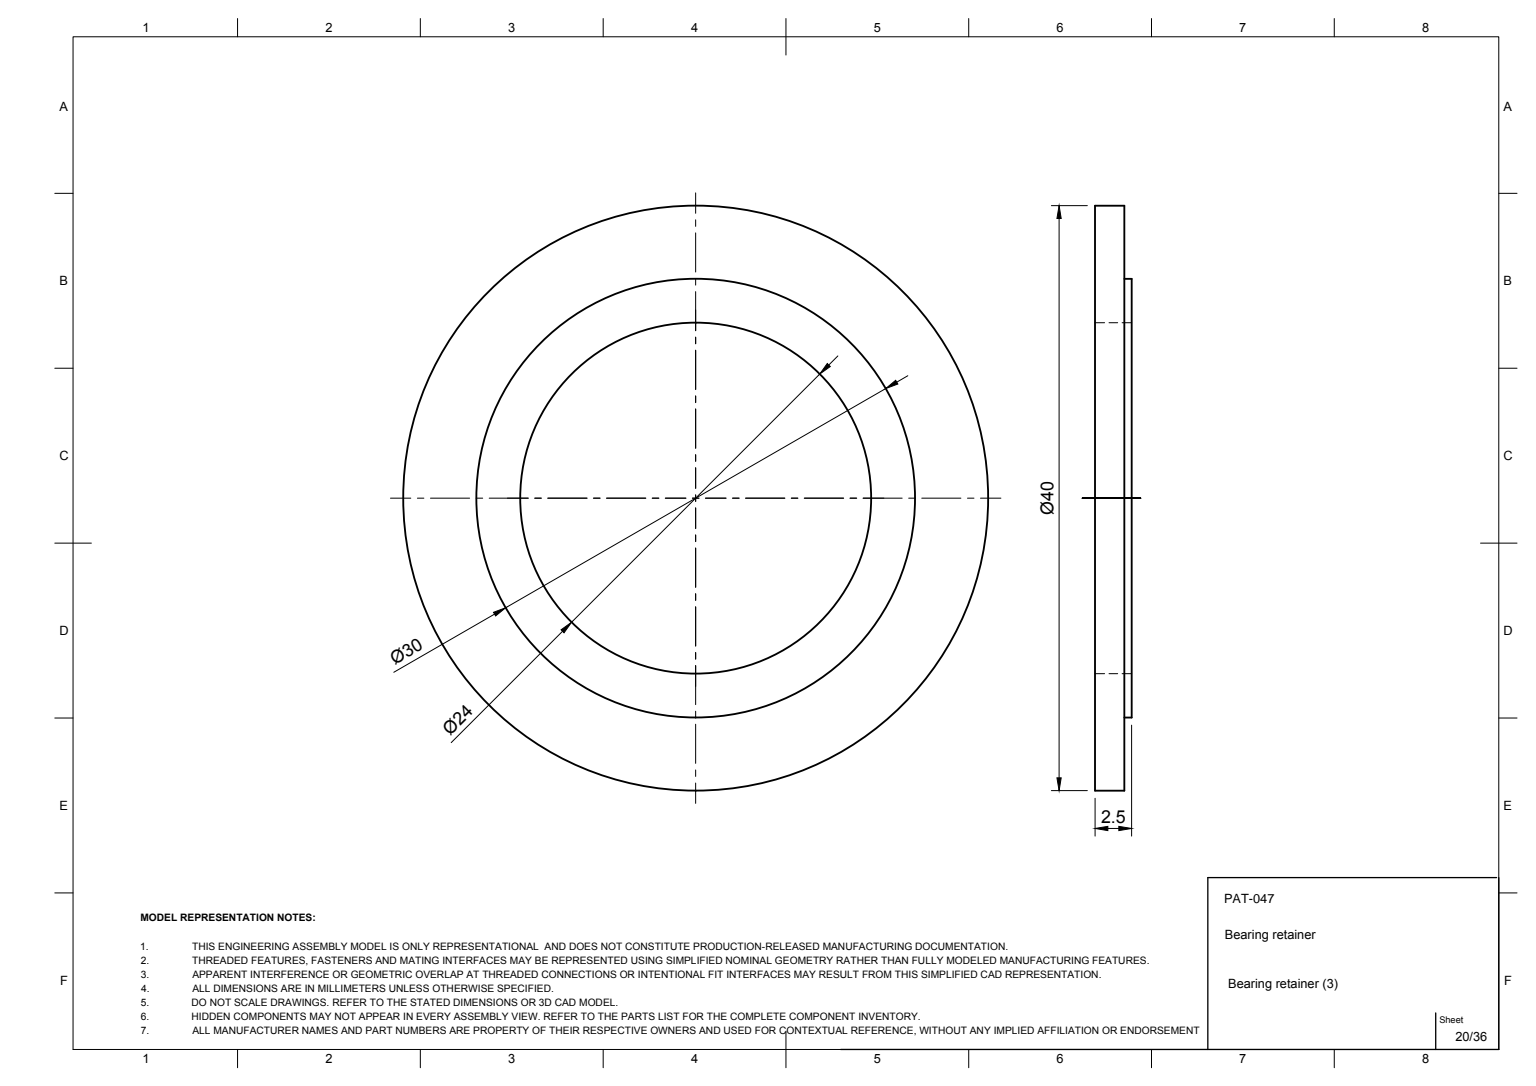
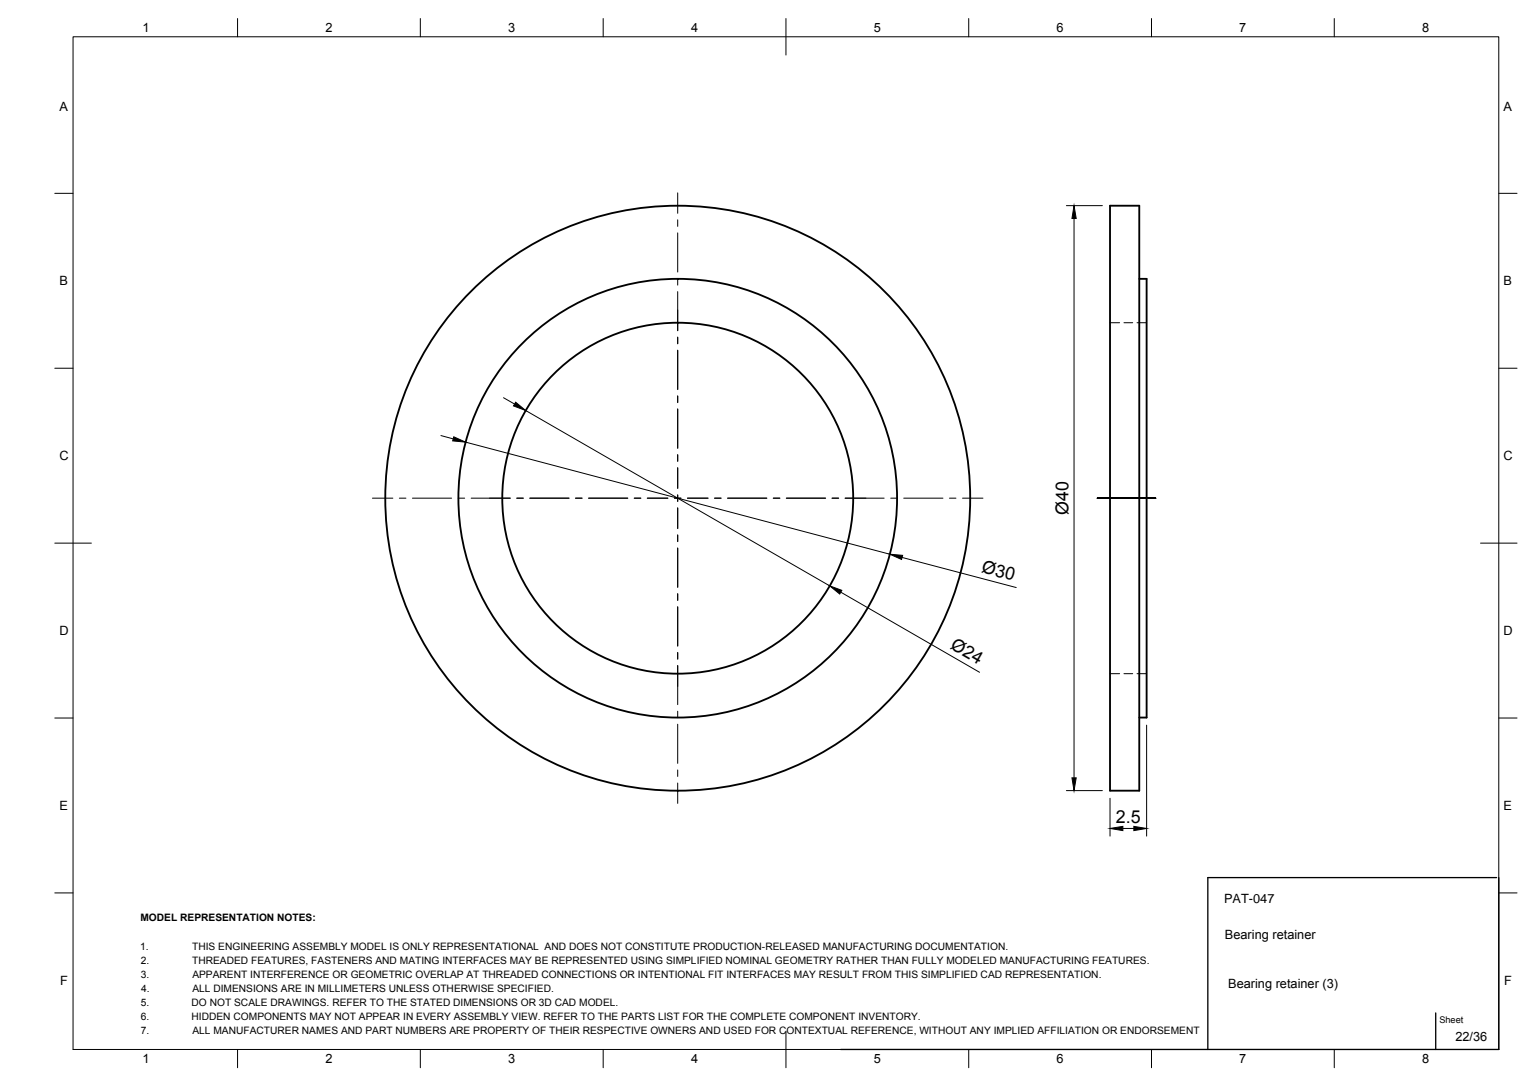
ISO-10303-21;
HEADER;
/* Generated by software containing ST-Developer
 * from STEP Tools, Inc. (www.steptools.com) 
 */

FILE_DESCRIPTION(
/* description */ ('Gravity roller conveyor section'),
/* implementation_level */ '2;1');

FILE_NAME(
/* name */ 'Bearing retainer.step',
/* time_stamp */ '2026-11-02T07:43:02-08:00',
/* author */ (''),
/* organization */ (''),
/* preprocessor_version */ 'ST-DEVELOPER v20.2',
/* originating_system */ 'Autodesk Translation Framework v15.17.0.0',
/* authorisation */ '');

FILE_SCHEMA (('AUTOMOTIVE_DESIGN { 1 0 10303 214 3 1 1 }'));
ENDSEC;

DATA;
#10=MECHANICAL_DESIGN_GEOMETRIC_PRESENTATION_REPRESENTATION('',(#545),#13821);
#477=SHAPE_REPRESENTATION_RELATIONSHIP('SRR','None',#14015,#511);
#511=ADVANCED_BREP_SHAPE_REPRESENTATION('',(#585),#13802);
#545=STYLED_ITEM('',(#14191),#585);
#585=MANIFOLD_SOLID_BREP('Body1',#7645);
#655=FACE_BOUND('',#1729,.T.);
#656=FACE_BOUND('',#1733,.T.);
#657=FACE_BOUND('',#1735,.T.);
#918=PLANE('',#8392);
#919=PLANE('',#8399);
#920=PLANE('',#8400);
#1262=FACE_OUTER_BOUND('',#1727,.T.);
#1263=FACE_OUTER_BOUND('',#1728,.T.);
#1264=FACE_OUTER_BOUND('',#1730,.T.);
#1265=FACE_OUTER_BOUND('',#1731,.T.);
#1266=FACE_OUTER_BOUND('',#1732,.T.);
#1267=FACE_OUTER_BOUND('',#1734,.T.);
#1727=EDGE_LOOP('',(#6492,#6493,#6494,#6495));
#1728=EDGE_LOOP('',(#6496));
#1729=EDGE_LOOP('',(#6497));
#1730=EDGE_LOOP('',(#6498,#6499,#6500,#6501));
#1731=EDGE_LOOP('',(#6502,#6503,#6504,#6505));
#1732=EDGE_LOOP('',(#6506));
#1733=EDGE_LOOP('',(#6507));
#1734=EDGE_LOOP('',(#6508));
#1735=EDGE_LOOP('',(#6509));
#2507=LINE('',#12595,#3225);
#2508=LINE('',#12602,#3226);
#2509=LINE('',#12608,#3227);
#3225=VECTOR('',#10072,1.5);
#3226=VECTOR('',#10081,1.2);
#3227=VECTOR('',#10088,2.);
#3440=CIRCLE('',#8390,1.5);
#3441=CIRCLE('',#8391,1.5);
#3442=CIRCLE('',#8393,1.2);
#3443=CIRCLE('',#8395,1.2);
#3444=CIRCLE('',#8397,2.);
#3445=CIRCLE('',#8398,2.);
#4018=VERTEX_POINT('',#12592);
#4019=VERTEX_POINT('',#12594);
#4020=VERTEX_POINT('',#12598);
#4021=VERTEX_POINT('',#12601);
#4022=VERTEX_POINT('',#12605);
#4023=VERTEX_POINT('',#12607);
#4883=EDGE_CURVE('',#4018,#4018,#3440,.T.);
#4884=EDGE_CURVE('',#4018,#4019,#2507,.T.);
#4885=EDGE_CURVE('',#4019,#4019,#3441,.T.);
#4886=EDGE_CURVE('',#4020,#4020,#3442,.T.);
#4887=EDGE_CURVE('',#4020,#4021,#2508,.T.);
#4888=EDGE_CURVE('',#4021,#4021,#3443,.T.);
#4889=EDGE_CURVE('',#4022,#4022,#3444,.T.);
#4890=EDGE_CURVE('',#4022,#4023,#2509,.T.);
#4891=EDGE_CURVE('',#4023,#4023,#3445,.T.);
#6492=ORIENTED_EDGE('',*,*,#4883,.F.);
#6493=ORIENTED_EDGE('',*,*,#4884,.T.);
#6494=ORIENTED_EDGE('',*,*,#4885,.F.);
#6495=ORIENTED_EDGE('',*,*,#4884,.F.);
#6496=ORIENTED_EDGE('',*,*,#4885,.T.);
#6497=ORIENTED_EDGE('',*,*,#4886,.T.);
#6498=ORIENTED_EDGE('',*,*,#4886,.F.);
#6499=ORIENTED_EDGE('',*,*,#4887,.T.);
#6500=ORIENTED_EDGE('',*,*,#4888,.T.);
#6501=ORIENTED_EDGE('',*,*,#4887,.F.);
#6502=ORIENTED_EDGE('',*,*,#4889,.F.);
#6503=ORIENTED_EDGE('',*,*,#4890,.T.);
#6504=ORIENTED_EDGE('',*,*,#4891,.T.);
#6505=ORIENTED_EDGE('',*,*,#4890,.F.);
#6506=ORIENTED_EDGE('',*,*,#4889,.T.);
#6507=ORIENTED_EDGE('',*,*,#4883,.T.);
#6508=ORIENTED_EDGE('',*,*,#4891,.F.);
#6509=ORIENTED_EDGE('',*,*,#4888,.F.);
#7161=CYLINDRICAL_SURFACE('',#8389,1.5);
#7162=CYLINDRICAL_SURFACE('',#8394,1.2);
#7163=CYLINDRICAL_SURFACE('',#8396,2.);
#7463=ADVANCED_FACE('',(#1262),#7161,.T.);
#7464=ADVANCED_FACE('',(#1263,#655),#918,.T.);
#7465=ADVANCED_FACE('',(#1264),#7162,.F.);
#7466=ADVANCED_FACE('',(#1265),#7163,.T.);
#7467=ADVANCED_FACE('',(#1266,#656),#919,.T.);
#7468=ADVANCED_FACE('',(#1267,#657),#920,.F.);
#7645=CLOSED_SHELL('',(#7463,#7464,#7465,#7466,#7467,#7468));
#8388=AXIS2_PLACEMENT_3D('',#12590,#10066,#10067);
#8389=AXIS2_PLACEMENT_3D('',#12591,#10068,#10069);
#8390=AXIS2_PLACEMENT_3D('',#12593,#10070,#10071);
#8391=AXIS2_PLACEMENT_3D('',#12596,#10073,#10074);
#8392=AXIS2_PLACEMENT_3D('',#12597,#10075,#10076);
#8393=AXIS2_PLACEMENT_3D('',#12599,#10077,#10078);
#8394=AXIS2_PLACEMENT_3D('',#12600,#10079,#10080);
#8395=AXIS2_PLACEMENT_3D('',#12603,#10082,#10083);
#8396=AXIS2_PLACEMENT_3D('',#12604,#10084,#10085);
#8397=AXIS2_PLACEMENT_3D('',#12606,#10086,#10087);
#8398=AXIS2_PLACEMENT_3D('',#12609,#10089,#10090);
#8399=AXIS2_PLACEMENT_3D('',#12610,#10091,#10092);
#8400=AXIS2_PLACEMENT_3D('',#12611,#10093,#10094);
#10066=DIRECTION('axis',(0.,0.,1.));
#10067=DIRECTION('refdir',(1.,0.,0.));
#10068=DIRECTION('center_axis',(0.,1.,0.));
#10069=DIRECTION('ref_axis',(1.,0.,0.));
#10070=DIRECTION('center_axis',(0.,-1.,0.));
#10071=DIRECTION('ref_axis',(1.,0.,0.));
#10072=DIRECTION('',(0.,1.,0.));
#10073=DIRECTION('center_axis',(0.,1.,0.));
#10074=DIRECTION('ref_axis',(1.,0.,0.));
#10075=DIRECTION('center_axis',(0.,1.,0.));
#10076=DIRECTION('ref_axis',(1.,0.,0.));
#10077=DIRECTION('center_axis',(0.,-1.,0.));
#10078=DIRECTION('ref_axis',(1.,0.,0.));
#10079=DIRECTION('center_axis',(0.,1.,0.));
#10080=DIRECTION('ref_axis',(1.,0.,0.));
#10081=DIRECTION('',(0.,-1.,0.));
#10082=DIRECTION('center_axis',(0.,-1.,0.));
#10083=DIRECTION('ref_axis',(1.,0.,0.));
#10084=DIRECTION('center_axis',(0.,1.,0.));
#10085=DIRECTION('ref_axis',(1.,0.,0.));
#10086=DIRECTION('center_axis',(0.,1.,0.));
#10087=DIRECTION('ref_axis',(1.,0.,0.));
#10088=DIRECTION('',(0.,-1.,0.));
#10089=DIRECTION('center_axis',(0.,1.,0.));
#10090=DIRECTION('ref_axis',(1.,0.,0.));
#10091=DIRECTION('center_axis',(0.,1.,0.));
#10092=DIRECTION('ref_axis',(1.,0.,0.));
#10093=DIRECTION('center_axis',(0.,1.,0.));
#10094=DIRECTION('ref_axis',(1.,0.,0.));
#12590=CARTESIAN_POINT('',(0.,0.,0.));
#12591=CARTESIAN_POINT('Origin',(3.,0.,8.));
#12592=CARTESIAN_POINT('',(1.5,0.,8.));
#12593=CARTESIAN_POINT('Origin',(3.,0.,8.));
#12594=CARTESIAN_POINT('',(1.5,0.05,8.));
#12595=CARTESIAN_POINT('',(1.5,0.,8.));
#12596=CARTESIAN_POINT('Origin',(3.,0.05,8.));
#12597=CARTESIAN_POINT('Origin',(3.,0.05,8.));
#12598=CARTESIAN_POINT('',(1.8,0.05,8.));
#12599=CARTESIAN_POINT('Origin',(3.,0.05,8.));
#12600=CARTESIAN_POINT('Origin',(3.,-0.2,8.));
#12601=CARTESIAN_POINT('',(1.8,-0.2,8.));
#12602=CARTESIAN_POINT('',(1.8,-0.2,8.));
#12603=CARTESIAN_POINT('Origin',(3.,-0.2,8.));
#12604=CARTESIAN_POINT('Origin',(3.,-0.2,8.));
#12605=CARTESIAN_POINT('',(1.,0.,8.));
#12606=CARTESIAN_POINT('Origin',(3.,0.,8.));
#12607=CARTESIAN_POINT('',(1.,-0.2,8.));
#12608=CARTESIAN_POINT('',(1.,-0.2,8.));
#12609=CARTESIAN_POINT('Origin',(3.,-0.2,8.));
#12610=CARTESIAN_POINT('Origin',(3.,0.,8.));
#12611=CARTESIAN_POINT('Origin',(3.,-0.2,8.));
#13763=UNCERTAINTY_MEASURE_WITH_UNIT(LENGTH_MEASURE(0.001),#13822,
'DISTANCE_ACCURACY_VALUE',
'Maximum model space distance between geometric entities at asserted c
onnectivities');
#13782=UNCERTAINTY_MEASURE_WITH_UNIT(LENGTH_MEASURE(0.001),#13822,
'DISTANCE_ACCURACY_VALUE',
'Maximum model space distance between geometric entities at asserted c
onnectivities');
#13802=(
GEOMETRIC_REPRESENTATION_CONTEXT(3)
GLOBAL_UNCERTAINTY_ASSIGNED_CONTEXT((#13763))
GLOBAL_UNIT_ASSIGNED_CONTEXT((#13822,#13824,#13825))
REPRESENTATION_CONTEXT('','3D')
);
#13821=(
GEOMETRIC_REPRESENTATION_CONTEXT(3)
GLOBAL_UNCERTAINTY_ASSIGNED_CONTEXT((#13782))
GLOBAL_UNIT_ASSIGNED_CONTEXT((#13822,#13824,#13825))
REPRESENTATION_CONTEXT('','3D')
);
#13822=(
LENGTH_UNIT()
NAMED_UNIT(*)
SI_UNIT(.CENTI.,.METRE.)
);
#13824=(
NAMED_UNIT(*)
PLANE_ANGLE_UNIT()
SI_UNIT($,.RADIAN.)
);
#13825=(
NAMED_UNIT(*)
SI_UNIT($,.STERADIAN.)
SOLID_ANGLE_UNIT()
);
#13845=SHAPE_DEFINITION_REPRESENTATION(#13883,#14015);
#13883=PRODUCT_DEFINITION_SHAPE('',$,#14054);
#14015=SHAPE_REPRESENTATION('',(#8388),#13802);
#14034=PRODUCT_DEFINITION_CONTEXT('part definition',#14150,'design');
#14054=PRODUCT_DEFINITION('Bearing retainer','Bearing retainer',#14092,
#14034);
#14092=PRODUCT_DEFINITION_FORMATION('',$,#14171);
#14150=APPLICATION_CONTEXT(
'Core Data for Automotive Mechanical Design Process');
#14151=PRODUCT_CONTEXT('part definition',#14150,'mechanical');
#14171=PRODUCT('Bearing retainer','Bearing retainer','Bearing retainer',
(#14151));
#14191=PRESENTATION_STYLE_ASSIGNMENT((#14196));
#14196=SURFACE_STYLE_USAGE(.BOTH.,#14201);
#14201=SURFACE_SIDE_STYLE('',(#14206));
#14206=SURFACE_STYLE_FILL_AREA(#14211);
#14211=FILL_AREA_STYLE('CAD Library Painted - Steel gray',(#14216));
#14216=FILL_AREA_STYLE_COLOUR('CAD Library Painted - Steel gray',#14221);
#14221=COLOUR_RGB('CAD Library Painted - Steel gray',0.592156862745098,
0.631372549019608,0.67843137254902);
ENDSEC;
END-ISO-10303-21;
